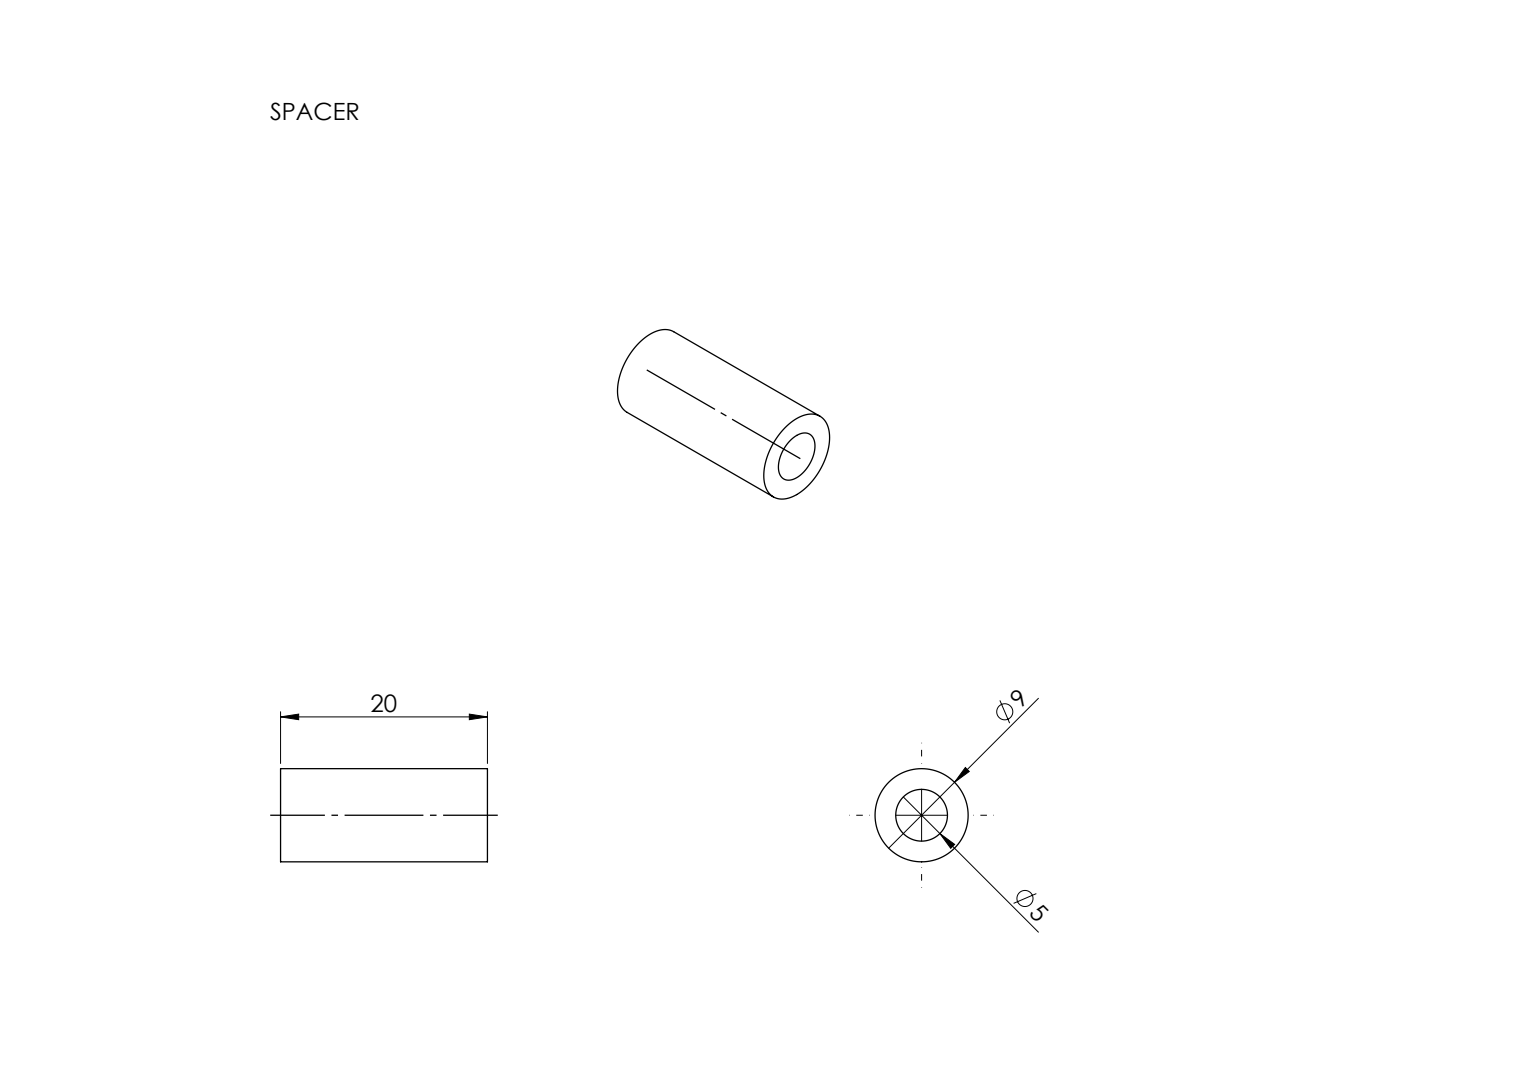
ISO-10303-21;
HEADER;
FILE_DESCRIPTION (('STEP AP214'),
    '1' );
FILE_NAME ('spacer.step',
    '2026-10-03T20:08:58',
    ( '' ),
    ( '' ),
    'SwSTEP 2.0',
    'SolidWorks 2026',
    '' );
FILE_SCHEMA (( 'AUTOMOTIVE_DESIGN' ));
ENDSEC;

DATA;
#9=AXIS2_PLACEMENT_3D ( 'NONE', #3779, #3718, #5895 ) ;
#33=DIRECTION ( 'NONE',  ( 1.000000000000000000, 1.081682119347366321E-16, -5.551115123125780237E-17 ) ) ;
#85=FACE_OUTER_BOUND ( 'NONE', #4807, .T. ) ;
#92=CARTESIAN_POINT ( 'NONE',  ( 40.00000000000006395, 1.290960574571364216E-15, -20.00000000000000000 ) ) ;
#144=VERTEX_POINT ( 'NONE', #12137 ) ;
#256=AXIS2_PLACEMENT_3D ( 'NONE', #10439, #11422, #1428 ) ;
#292=AXIS2_PLACEMENT_3D ( 'NONE', #6749, #3786, #3026 ) ;
#326=EDGE_CURVE ( 'NONE', #1272, #144, #5806, .T. ) ;
#391=STYLED_ITEM ( 'NONE', ( #419 ), #1696 ) ;
#419=PRESENTATION_STYLE_ASSIGNMENT (( #10127 ) ) ;
#453=DIRECTION ( 'NONE',  ( -1.000000000000000000, -1.081682119347366444E-16, 5.551115123125780237E-17 ) ) ;
#480=FILL_AREA_STYLE ('',( #5374 ) ) ;
#517=PRODUCT_DEFINITION_SHAPE ( 'NONE', 'NONE',  #7290 ) ;
#632=COLOUR_RGB ( '', 0.66274510, 0.83137255, 0.94901961) ;
#777=CARTESIAN_POINT ( 'NONE',  ( 40.00000000000006395, -2.499999999999997335, -20.00000000000000000 ) ) ;
#848=FACE_OUTER_BOUND ( 'NONE', #7283, .T. ) ;
#995=PRODUCT_CONTEXT ( 'NONE', #12106, 'mechanical' ) ;
#1096=VECTOR ( 'NONE', #6134, 1000.000000000000000 ) ;
#1158=CARTESIAN_POINT ( 'NONE',  ( 40.00000000000006395, 1.290960574571364216E-15, -20.00000000000000000 ) ) ;
#1186=SHAPE_DEFINITION_REPRESENTATION ( #517, #3471 ) ;
#1225=CYLINDRICAL_SURFACE ( 'NONE', #5852, 2.499999999999998668 ) ;
#1238=AXIS2_PLACEMENT_3D ( 'NONE', #92, #33, #10841 ) ;
#1253=CYLINDRICAL_SURFACE ( 'NONE', #10328, 2.499999999999998668 ) ;
#1267=ADVANCED_FACE ( 'NONE', ( #85 ), #10767, .T. ) ;
#1272=VERTEX_POINT ( 'NONE', #2084 ) ;
#1289=CARTESIAN_POINT ( 'NONE',  ( 40.00000000000006395, 1.290960574571364216E-15, -20.00000000000000000 ) ) ;
#1329=ORIENTED_EDGE ( 'NONE', *, *, #3041, .F. ) ;
#1356=EDGE_CURVE ( 'NONE', #2130, #6863, #7172, .T. ) ;
#1358=( NAMED_UNIT ( * ) PLANE_ANGLE_UNIT ( ) SI_UNIT ( $, .RADIAN. ) );
#1418=CARTESIAN_POINT ( 'NONE',  ( 40.00000000000006395, 1.290960574571364216E-15, -20.00000000000000000 ) ) ;
#1428=DIRECTION ( 'NONE',  ( 0.000000000000000000, 1.000000000000000000, 0.000000000000000000 ) ) ;
#1435=CIRCLE ( 'NONE', #8641, 4.499999999999999112 ) ;
#1612=AXIS2_PLACEMENT_3D ( 'NONE', #11456, #8542, #2573 ) ;
#1683=EDGE_CURVE ( 'NONE', #5519, #3706, #8079, .T. ) ;
#1688=DIRECTION ( 'NONE',  ( -1.000000000000000000, -1.081682119347366444E-16, 5.551115123125780237E-17 ) ) ;
#1696=MANIFOLD_SOLID_BREP ( 'Extrude-Thin1', #2109 ) ;
#1874=DIRECTION ( 'NONE',  ( 0.000000000000000000, -1.000000000000000000, 0.000000000000000000 ) ) ;
#2037=MECHANICAL_DESIGN_GEOMETRIC_PRESENTATION_REPRESENTATION('',(#391),#6977);
#2084=CARTESIAN_POINT ( 'NONE',  ( 20.00000000000006750, -2.500000000000000000, -20.00000000000000000 ) ) ;
#2109=CLOSED_SHELL ( 'NONE', ( #3239, #7662, #9087, #11025, #1267, #7819 ) ) ;
#2130=VERTEX_POINT ( 'NONE', #777 ) ;
#2189=EDGE_CURVE ( 'NONE', #11297, #3706, #10268, .T. ) ;
#2338=DIRECTION ( 'NONE',  ( 1.000000000000000000, 1.081682119347366321E-16, -5.551115123125780237E-17 ) ) ;
#2342=( NAMED_UNIT ( * ) SI_UNIT ( $, .STERADIAN. ) SOLID_ANGLE_UNIT ( ) );
#2349=EDGE_CURVE ( 'NONE', #5519, #9099, #1435, .T. ) ;
#2366=( LENGTH_UNIT ( ) NAMED_UNIT ( * ) SI_UNIT ( .MILLI., .METRE. ) );
#2399=PLANE ( 'NONE',  #4713 ) ;
#2425=SURFACE_SIDE_STYLE ('',( #10981 ) ) ;
#2482=AXIS2_PLACEMENT_3D ( 'NONE', #3935, #3996, #1874 ) ;
#2517=UNCERTAINTY_MEASURE_WITH_UNIT (LENGTH_MEASURE( 1.000000000000000082E-05 ), #10299, 'distance_accuracy_value', 'NONE');
#2573=DIRECTION ( 'NONE',  ( 0.000000000000000000, 1.000000000000000000, 0.000000000000000000 ) ) ;
#2588=PRODUCT ( 'spacer', 'spacer', '', ( #995 ) ) ;
#2662=AXIS2_PLACEMENT_3D ( 'NONE', #5050, #3008, #4798 ) ;
#2872=FACE_BOUND ( 'NONE', #7830, .T. ) ;
#3008=DIRECTION ( 'NONE',  ( -1.000000000000000000, -1.081682119347366444E-16, 5.551115123125780237E-17 ) ) ;
#3018=ORIENTED_EDGE ( 'NONE', *, *, #3041, .T. ) ;
#3026=DIRECTION ( 'NONE',  ( 0.000000000000000000, 1.000000000000000000, 0.000000000000000000 ) ) ;
#3041=EDGE_CURVE ( 'NONE', #144, #1272, #5845, .T. ) ;
#3118=DIRECTION ( 'NONE',  ( 0.000000000000000000, -1.000000000000000000, 0.000000000000000000 ) ) ;
#3148=ORIENTED_EDGE ( 'NONE', *, *, #8827, .F. ) ;
#3192=( LENGTH_UNIT ( ) NAMED_UNIT ( * ) SI_UNIT ( .MILLI., .METRE. ) );
#3201=EDGE_CURVE ( 'NONE', #6863, #2130, #7275, .T. ) ;
#3239=ADVANCED_FACE ( 'NONE', ( #10067 ), #1253, .F. ) ;
#3278=DIRECTION ( 'NONE',  ( -1.000000000000000000, -1.081682119347366444E-16, 5.551115123125780237E-17 ) ) ;
#3348=ORIENTED_EDGE ( 'NONE', *, *, #5521, .F. ) ;
#3380=FILL_AREA_STYLE ('',( #3501 ) ) ;
#3420=ORIENTED_EDGE ( 'NONE', *, *, #1683, .F. ) ;
#3471=SHAPE_REPRESENTATION ( 'spacer', ( #12422 ), #4543 ) ;
#3501=FILL_AREA_STYLE_COLOUR ( '', #632 ) ;
#3577=EDGE_CURVE ( 'NONE', #9099, #11297, #4012, .T. ) ;
#3656=FACE_BOUND ( 'NONE', #7270, .T. ) ;
#3706=VERTEX_POINT ( 'NONE', #9855 ) ;
#3718=DIRECTION ( 'NONE',  ( 1.000000000000000000, 1.081682119347366321E-16, -5.551115123125780237E-17 ) ) ;
#3779=CARTESIAN_POINT ( 'NONE',  ( 20.00000000000006750, -8.724036641233686229E-16, -20.00000000000000000 ) ) ;
#3786=DIRECTION ( 'NONE',  ( 1.000000000000000000, 1.081682119347366321E-16, -5.551115123125780237E-17 ) ) ;
#3926=EDGE_CURVE ( 'NONE', #2130, #1272, #10504, .T. ) ;
#3935=CARTESIAN_POINT ( 'NONE',  ( 20.00000000000006750, -8.724036641233686229E-16, -20.00000000000000000 ) ) ;
#3996=DIRECTION ( 'NONE',  ( 1.000000000000000000, 1.081682119347366321E-16, -5.551115123125780237E-17 ) ) ;
#4004=AXIS2_PLACEMENT_3D ( 'NONE', #9907, #4783, #7805 ) ;
#4009=ORIENTED_EDGE ( 'NONE', *, *, #326, .T. ) ;
#4012=LINE ( 'NONE', #9918, #1096 ) ;
#4029=DIRECTION ( 'NONE',  ( 1.000000000000000000, 1.081682119347366321E-16, -5.551115123125780237E-17 ) ) ;
#4177=AXIS2_PLACEMENT_3D ( 'NONE', #6089, #4029, #8921 ) ;
#4234=ORIENTED_EDGE ( 'NONE', *, *, #1356, .F. ) ;
#4332=STYLED_ITEM ( 'NONE', ( #7424 ), #4339 ) ;
#4339=ADVANCED_BREP_SHAPE_REPRESENTATION ( '', ( #1696, #12422 ), #4543 ) ;
#4387=CARTESIAN_POINT ( 'NONE',  ( 40.00000000000006395, 4.500000000000000000, -20.00000000000000000 ) ) ;
#4406=CARTESIAN_POINT ( 'NONE',  ( 20.00000000000006750, 4.499999999999998224, -20.00000000000000000 ) ) ;
#4543=( GEOMETRIC_REPRESENTATION_CONTEXT ( 3 ) GLOBAL_UNCERTAINTY_ASSIGNED_CONTEXT ( ( #10481 ) ) GLOBAL_UNIT_ASSIGNED_CONTEXT ( ( #3192, #9086, #2342 ) ) REPRESENTATION_CONTEXT ( 'NONE', 'WORKASPACE' ) );
#4544=CIRCLE ( 'NONE', #1238, 4.499999999999999112 ) ;
#4713=AXIS2_PLACEMENT_3D ( 'NONE', #1418, #2338, #7102 ) ;
#4783=DIRECTION ( 'NONE',  ( -1.000000000000000000, -1.081682119347366444E-16, 5.551115123125780237E-17 ) ) ;
#4798=DIRECTION ( 'NONE',  ( 0.000000000000000000, -1.000000000000000000, 0.000000000000000000 ) ) ;
#4807=EDGE_LOOP ( 'NONE', ( #8805, #7328, #5014, #8475 ) ) ;
#5014=ORIENTED_EDGE ( 'NONE', *, *, #1683, .T. ) ;
#5028=ORIENTED_EDGE ( 'NONE', *, *, #3926, .T. ) ;
#5050=CARTESIAN_POINT ( 'NONE',  ( 40.00000000000006395, 1.290960574571364216E-15, -20.00000000000000000 ) ) ;
#5124=( NAMED_UNIT ( * ) SI_UNIT ( $, .STERADIAN. ) SOLID_ANGLE_UNIT ( ) );
#5193=CARTESIAN_POINT ( 'NONE',  ( 40.00000000000006395, 1.290960574571364216E-15, -20.00000000000000000 ) ) ;
#5265=APPLICATION_CONTEXT ( 'automotive_design' ) ;
#5288=PRODUCT_DEFINITION_FORMATION_WITH_SPECIFIED_SOURCE ( 'ANY', '', #2588, .NOT_KNOWN. ) ;
#5374=FILL_AREA_STYLE_COLOUR ( '', #5938 ) ;
#5519=VERTEX_POINT ( 'NONE', #9266 ) ;
#5521=EDGE_CURVE ( 'NONE', #6863, #144, #6451, .T. ) ;
#5707=CARTESIAN_POINT ( 'NONE',  ( 0.000000000000000000, 0.000000000000000000, 0.000000000000000000 ) ) ;
#5806=CIRCLE ( 'NONE', #256, 2.499999999999998668 ) ;
#5845=CIRCLE ( 'NONE', #292, 2.499999999999998668 ) ;
#5852=AXIS2_PLACEMENT_3D ( 'NONE', #1289, #11994, #3118 ) ;
#5895=DIRECTION ( 'NONE',  ( -1.081682119347366321E-16, 1.000000000000000000, 0.000000000000000000 ) ) ;
#5929=CYLINDRICAL_SURFACE ( 'NONE', #4004, 4.499999999999999112 ) ;
#5938=COLOUR_RGB ( '', 0.66274510, 0.83137255, 0.94901961) ;
#6089=CARTESIAN_POINT ( 'NONE',  ( 40.00000000000006395, 1.290960574571364216E-15, -20.00000000000000000 ) ) ;
#6134=DIRECTION ( 'NONE',  ( -1.000000000000000000, -1.081682119347366444E-16, 5.551115123125780237E-17 ) ) ;
#6428=DIRECTION ( 'NONE',  ( 1.000000000000000000, 0.000000000000000000, 0.000000000000000000 ) ) ;
#6451=LINE ( 'NONE', #10359, #8557 ) ;
#6459=VECTOR ( 'NONE', #1688, 1000.000000000000000 ) ;
#6523=SHAPE_REPRESENTATION_RELATIONSHIP ( 'NONE' , 'NONE' ,  #3471, #4339 ) ;
#6664=CARTESIAN_POINT ( 'NONE',  ( 20.00000000000006750, -8.724036641233686229E-16, -20.00000000000000000 ) ) ;
#6749=CARTESIAN_POINT ( 'NONE',  ( 20.00000000000006750, -8.724036641233686229E-16, -20.00000000000000000 ) ) ;
#6863=VERTEX_POINT ( 'NONE', #9753 ) ;
#6891=EDGE_LOOP ( 'NONE', ( #3148, #8538 ) ) ;
#6977=( GEOMETRIC_REPRESENTATION_CONTEXT ( 3 ) GLOBAL_UNCERTAINTY_ASSIGNED_CONTEXT ( ( #12525 ) ) GLOBAL_UNIT_ASSIGNED_CONTEXT ( ( #2366, #8144, #5124 ) ) REPRESENTATION_CONTEXT ( 'NONE', 'WORKASPACE' ) );
#7087=PRODUCT_DEFINITION_CONTEXT ( 'detailed design', #5265, 'design' ) ;
#7102=DIRECTION ( 'NONE',  ( -1.081682119347366321E-16, 1.000000000000000000, 0.000000000000000000 ) ) ;
#7172=CIRCLE ( 'NONE', #1612, 2.499999999999998668 ) ;
#7191=DIRECTION ( 'NONE',  ( 0.000000000000000000, -1.000000000000000000, 0.000000000000000000 ) ) ;
#7270=EDGE_LOOP ( 'NONE', ( #4009, #3018 ) ) ;
#7275=CIRCLE ( 'NONE', #4177, 2.499999999999998668 ) ;
#7283=EDGE_LOOP ( 'NONE', ( #12294, #10776, #9997, #3420 ) ) ;
#7290=PRODUCT_DEFINITION ( 'UNKNOWN', '', #5288, #7087 ) ;
#7298=EDGE_LOOP ( 'NONE', ( #3348, #10484, #5028, #1329 ) ) ;
#7328=ORIENTED_EDGE ( 'NONE', *, *, #2349, .F. ) ;
#7392=DIRECTION ( 'NONE',  ( 0.000000000000000000, 0.000000000000000000, 1.000000000000000000 ) ) ;
#7424=PRESENTATION_STYLE_ASSIGNMENT (( #12259 ) ) ;
#7527=ORIENTED_EDGE ( 'NONE', *, *, #10033, .T. ) ;
#7662=ADVANCED_FACE ( 'NONE', ( #848 ), #5929, .T. ) ;
#7805=DIRECTION ( 'NONE',  ( 0.000000000000000000, -1.000000000000000000, 0.000000000000000000 ) ) ;
#7819=ADVANCED_FACE ( 'NONE', ( #12061 ), #1225, .F. ) ;
#7830=EDGE_LOOP ( 'NONE', ( #4234, #12300 ) ) ;
#8079=LINE ( 'NONE', #10249, #9417 ) ;
#8099=CIRCLE ( 'NONE', #12443, 4.499999999999999112 ) ;
#8144=( NAMED_UNIT ( * ) PLANE_ANGLE_UNIT ( ) SI_UNIT ( $, .RADIAN. ) );
#8188=SURFACE_STYLE_FILL_AREA ( #3380 ) ;
#8475=ORIENTED_EDGE ( 'NONE', *, *, #8827, .T. ) ;
#8538=ORIENTED_EDGE ( 'NONE', *, *, #2189, .F. ) ;
#8542=DIRECTION ( 'NONE',  ( 1.000000000000000000, 1.081682119347366321E-16, -5.551115123125780237E-17 ) ) ;
#8557=VECTOR ( 'NONE', #453, 1000.000000000000000 ) ;
#8641=AXIS2_PLACEMENT_3D ( 'NONE', #1158, #11147, #9138 ) ;
#8668=FACE_OUTER_BOUND ( 'NONE', #6891, .T. ) ;
#8714=FACE_OUTER_BOUND ( 'NONE', #12510, .T. ) ;
#8805=ORIENTED_EDGE ( 'NONE', *, *, #3577, .F. ) ;
#8827=EDGE_CURVE ( 'NONE', #3706, #11297, #8099, .T. ) ;
#8853=( GEOMETRIC_REPRESENTATION_CONTEXT ( 3 ) GLOBAL_UNCERTAINTY_ASSIGNED_CONTEXT ( ( #2517 ) ) GLOBAL_UNIT_ASSIGNED_CONTEXT ( ( #10299, #1358, #12132 ) ) REPRESENTATION_CONTEXT ( 'NONE', 'WORKASPACE' ) );
#8921=DIRECTION ( 'NONE',  ( 0.000000000000000000, 1.000000000000000000, 0.000000000000000000 ) ) ;
#8979=EDGE_LOOP ( 'NONE', ( #11563, #10536, #9915, #11858 ) ) ;
#9086=( NAMED_UNIT ( * ) PLANE_ANGLE_UNIT ( ) SI_UNIT ( $, .RADIAN. ) );
#9087=ADVANCED_FACE ( 'NONE', ( #8714, #2872 ), #2399, .T. ) ;
#9099=VERTEX_POINT ( 'NONE', #4387 ) ;
#9138=DIRECTION ( 'NONE',  ( 0.000000000000000000, -1.000000000000000000, 0.000000000000000000 ) ) ;
#9266=CARTESIAN_POINT ( 'NONE',  ( 40.00000000000006395, -4.499999999999998224, -20.00000000000000000 ) ) ;
#9417=VECTOR ( 'NONE', #12024, 1000.000000000000000 ) ;
#9753=CARTESIAN_POINT ( 'NONE',  ( 40.00000000000006395, 2.500000000000000000, -20.00000000000000000 ) ) ;
#9855=CARTESIAN_POINT ( 'NONE',  ( 20.00000000000006750, -4.500000000000000000, -20.00000000000000000 ) ) ;
#9907=CARTESIAN_POINT ( 'NONE',  ( 40.00000000000006395, 1.290960574571364216E-15, -20.00000000000000000 ) ) ;
#9915=ORIENTED_EDGE ( 'NONE', *, *, #326, .F. ) ;
#9918=CARTESIAN_POINT ( 'NONE',  ( 40.00000000000006395, 4.500000000000000000, -20.00000000000000000 ) ) ;
#9997=ORIENTED_EDGE ( 'NONE', *, *, #2189, .T. ) ;
#10033=EDGE_CURVE ( 'NONE', #9099, #5519, #4544, .T. ) ;
#10067=FACE_OUTER_BOUND ( 'NONE', #8979, .T. ) ;
#10127=SURFACE_STYLE_USAGE ( .BOTH. , #2425 ) ;
#10249=CARTESIAN_POINT ( 'NONE',  ( 40.00000000000006395, -4.499999999999998224, -20.00000000000000000 ) ) ;
#10268=CIRCLE ( 'NONE', #2482, 4.499999999999999112 ) ;
#10299=( LENGTH_UNIT ( ) NAMED_UNIT ( * ) SI_UNIT ( .MILLI., .METRE. ) );
#10328=AXIS2_PLACEMENT_3D ( 'NONE', #5193, #3278, #7191 ) ;
#10359=CARTESIAN_POINT ( 'NONE',  ( 40.00000000000006395, 2.500000000000000000, -20.00000000000000000 ) ) ;
#10439=CARTESIAN_POINT ( 'NONE',  ( 20.00000000000006750, -8.724036641233686229E-16, -20.00000000000000000 ) ) ;
#10481=UNCERTAINTY_MEASURE_WITH_UNIT (LENGTH_MEASURE( 1.000000000000000082E-05 ), #3192, 'distance_accuracy_value', 'NONE');
#10484=ORIENTED_EDGE ( 'NONE', *, *, #3201, .T. ) ;
#10504=LINE ( 'NONE', #11912, #6459 ) ;
#10536=ORIENTED_EDGE ( 'NONE', *, *, #5521, .T. ) ;
#10569=DIRECTION ( 'NONE',  ( 0.000000000000000000, -1.000000000000000000, 0.000000000000000000 ) ) ;
#10767=CYLINDRICAL_SURFACE ( 'NONE', #2662, 4.499999999999999112 ) ;
#10776=ORIENTED_EDGE ( 'NONE', *, *, #3577, .T. ) ;
#10841=DIRECTION ( 'NONE',  ( 0.000000000000000000, -1.000000000000000000, 0.000000000000000000 ) ) ;
#10981=SURFACE_STYLE_FILL_AREA ( #480 ) ;
#11025=ADVANCED_FACE ( 'NONE', ( #8668, #3656 ), #12611, .F. ) ;
#11147=DIRECTION ( 'NONE',  ( 1.000000000000000000, 1.081682119347366321E-16, -5.551115123125780237E-17 ) ) ;
#11297=VERTEX_POINT ( 'NONE', #4406 ) ;
#11333=MECHANICAL_DESIGN_GEOMETRIC_PRESENTATION_REPRESENTATION('',(#4332),#8853);
#11422=DIRECTION ( 'NONE',  ( 1.000000000000000000, 1.081682119347366321E-16, -5.551115123125780237E-17 ) ) ;
#11456=CARTESIAN_POINT ( 'NONE',  ( 40.00000000000006395, 1.290960574571364216E-15, -20.00000000000000000 ) ) ;
#11563=ORIENTED_EDGE ( 'NONE', *, *, #1356, .T. ) ;
#11858=ORIENTED_EDGE ( 'NONE', *, *, #3926, .F. ) ;
#11912=CARTESIAN_POINT ( 'NONE',  ( 40.00000000000006395, -2.499999999999997335, -20.00000000000000000 ) ) ;
#11994=DIRECTION ( 'NONE',  ( -1.000000000000000000, -1.081682119347366444E-16, 5.551115123125780237E-17 ) ) ;
#12024=DIRECTION ( 'NONE',  ( -1.000000000000000000, -1.081682119347366444E-16, 5.551115123125780237E-17 ) ) ;
#12061=FACE_OUTER_BOUND ( 'NONE', #7298, .T. ) ;
#12098=ORIENTED_EDGE ( 'NONE', *, *, #2349, .T. ) ;
#12106=APPLICATION_CONTEXT ( 'automotive_design' ) ;
#12132=( NAMED_UNIT ( * ) SI_UNIT ( $, .STERADIAN. ) SOLID_ANGLE_UNIT ( ) );
#12137=CARTESIAN_POINT ( 'NONE',  ( 20.00000000000006750, 2.499999999999997780, -20.00000000000000000 ) ) ;
#12199=SURFACE_SIDE_STYLE ('',( #8188 ) ) ;
#12259=SURFACE_STYLE_USAGE ( .BOTH. , #12199 ) ;
#12294=ORIENTED_EDGE ( 'NONE', *, *, #10033, .F. ) ;
#12300=ORIENTED_EDGE ( 'NONE', *, *, #3201, .F. ) ;
#12422=AXIS2_PLACEMENT_3D ( 'NONE', #5707, #7392, #6428 ) ;
#12443=AXIS2_PLACEMENT_3D ( 'NONE', #6664, #12591, #10569 ) ;
#12510=EDGE_LOOP ( 'NONE', ( #12098, #7527 ) ) ;
#12525=UNCERTAINTY_MEASURE_WITH_UNIT (LENGTH_MEASURE( 1.000000000000000082E-05 ), #2366, 'distance_accuracy_value', 'NONE');
#12591=DIRECTION ( 'NONE',  ( 1.000000000000000000, 1.081682119347366321E-16, -5.551115123125780237E-17 ) ) ;
#12611=PLANE ( 'NONE',  #9 ) ;
ENDSEC;
END-ISO-10303-21;
